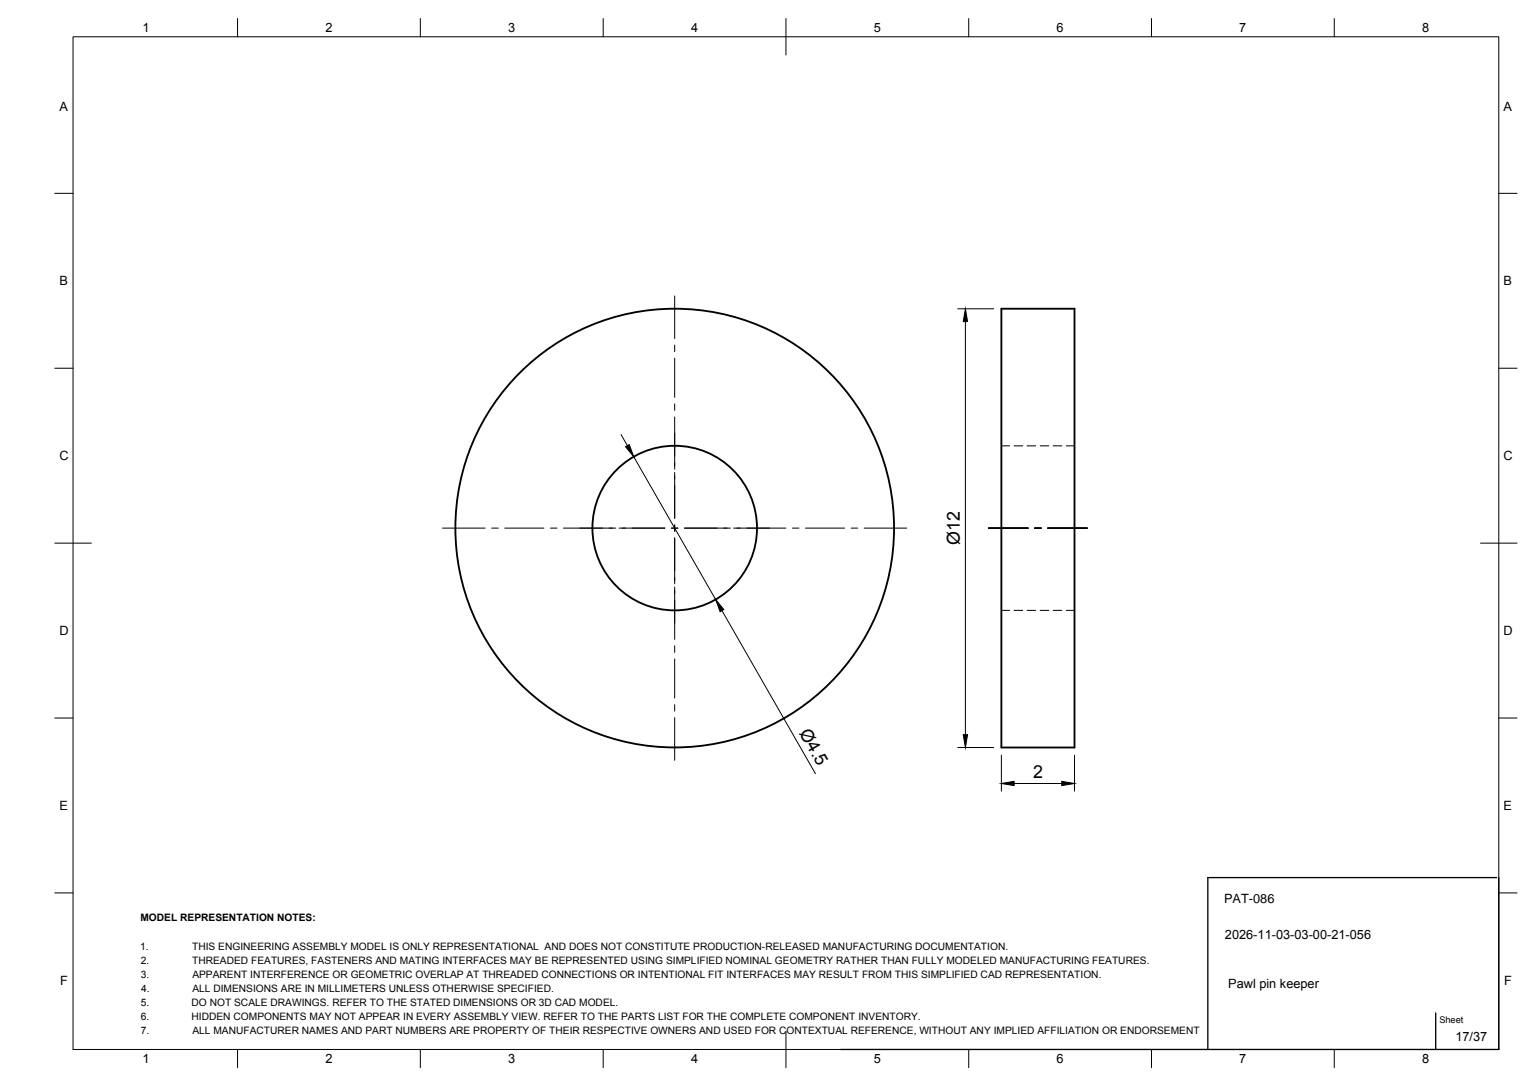
ISO-10303-21;
HEADER;
/* Generated by software containing ST-Developer
 * from STEP Tools, Inc. (www.steptools.com) 
 */

FILE_DESCRIPTION(
/* description */ ('Ratchet and pawl hand winch drum'),
/* implementation_level */ '2;1');

FILE_NAME(
/* name */ 'Pawl pin keeper.step',
/* time_stamp */ '2026-10-27T12:42:58-07:00',
/* author */ (''),
/* organization */ (''),
/* preprocessor_version */ 'ST-DEVELOPER v20.2',
/* originating_system */ 'Autodesk Translation Framework v15.17.0.0',
/* authorisation */ '');

FILE_SCHEMA (('AUTOMOTIVE_DESIGN { 1 0 10303 214 3 1 1 }'));
ENDSEC;

DATA;
#10=MECHANICAL_DESIGN_GEOMETRIC_PRESENTATION_REPRESENTATION('',(#401),#11801);
#333=SHAPE_REPRESENTATION_RELATIONSHIP('SRR','None',#11959,#367);
#367=ADVANCED_BREP_SHAPE_REPRESENTATION('',(#436),#11776);
#401=STYLED_ITEM('',(#12213),#436);
#436=MANIFOLD_SOLID_BREP('Body1',#6278);
#527=FACE_BOUND('',#1379,.T.);
#528=FACE_BOUND('',#1381,.T.);
#664=PLANE('',#6901);
#665=PLANE('',#6902);
#949=FACE_OUTER_BOUND('',#1376,.T.);
#950=FACE_OUTER_BOUND('',#1377,.T.);
#951=FACE_OUTER_BOUND('',#1378,.T.);
#952=FACE_OUTER_BOUND('',#1380,.T.);
#1376=EDGE_LOOP('',(#4691,#4692,#4693,#4694));
#1377=EDGE_LOOP('',(#4695,#4696,#4697,#4698));
#1378=EDGE_LOOP('',(#4699));
#1379=EDGE_LOOP('',(#4700));
#1380=EDGE_LOOP('',(#4701));
#1381=EDGE_LOOP('',(#4702));
#1827=LINE('',#9725,#2338);
#1828=LINE('',#9731,#2339);
#2338=VECTOR('',#7924,0.225);
#2339=VECTOR('',#7931,0.6);
#2811=CIRCLE('',#6896,0.225);
#2812=CIRCLE('',#6897,0.225);
#2813=CIRCLE('',#6899,0.6);
#2814=CIRCLE('',#6900,0.6);
#3090=VERTEX_POINT('',#9722);
#3091=VERTEX_POINT('',#9724);
#3092=VERTEX_POINT('',#9728);
#3093=VERTEX_POINT('',#9730);
#3689=EDGE_CURVE('',#3090,#3090,#2811,.T.);
#3690=EDGE_CURVE('',#3090,#3091,#1827,.T.);
#3691=EDGE_CURVE('',#3091,#3091,#2812,.T.);
#3692=EDGE_CURVE('',#3092,#3092,#2813,.T.);
#3693=EDGE_CURVE('',#3092,#3093,#1828,.T.);
#3694=EDGE_CURVE('',#3093,#3093,#2814,.T.);
#4691=ORIENTED_EDGE('',*,*,#3689,.F.);
#4692=ORIENTED_EDGE('',*,*,#3690,.T.);
#4693=ORIENTED_EDGE('',*,*,#3691,.T.);
#4694=ORIENTED_EDGE('',*,*,#3690,.F.);
#4695=ORIENTED_EDGE('',*,*,#3692,.F.);
#4696=ORIENTED_EDGE('',*,*,#3693,.T.);
#4697=ORIENTED_EDGE('',*,*,#3694,.T.);
#4698=ORIENTED_EDGE('',*,*,#3693,.F.);
#4699=ORIENTED_EDGE('',*,*,#3692,.T.);
#4700=ORIENTED_EDGE('',*,*,#3689,.T.);
#4701=ORIENTED_EDGE('',*,*,#3694,.F.);
#4702=ORIENTED_EDGE('',*,*,#3691,.F.);
#5853=CYLINDRICAL_SURFACE('',#6895,0.225);
#5854=CYLINDRICAL_SURFACE('',#6898,0.6);
#6019=ADVANCED_FACE('',(#949),#5853,.F.);
#6020=ADVANCED_FACE('',(#950),#5854,.T.);
#6021=ADVANCED_FACE('',(#951,#527),#664,.T.);
#6022=ADVANCED_FACE('',(#952,#528),#665,.F.);
#6278=CLOSED_SHELL('',(#6019,#6020,#6021,#6022));
#6894=AXIS2_PLACEMENT_3D('',#9720,#7918,#7919);
#6895=AXIS2_PLACEMENT_3D('',#9721,#7920,#7921);
#6896=AXIS2_PLACEMENT_3D('',#9723,#7922,#7923);
#6897=AXIS2_PLACEMENT_3D('',#9726,#7925,#7926);
#6898=AXIS2_PLACEMENT_3D('',#9727,#7927,#7928);
#6899=AXIS2_PLACEMENT_3D('',#9729,#7929,#7930);
#6900=AXIS2_PLACEMENT_3D('',#9732,#7932,#7933);
#6901=AXIS2_PLACEMENT_3D('',#9733,#7934,#7935);
#6902=AXIS2_PLACEMENT_3D('',#9734,#7936,#7937);
#7918=DIRECTION('axis',(0.,0.,1.));
#7919=DIRECTION('refdir',(1.,0.,0.));
#7920=DIRECTION('center_axis',(0.,1.,0.));
#7921=DIRECTION('ref_axis',(1.,0.,0.));
#7922=DIRECTION('center_axis',(0.,-1.,0.));
#7923=DIRECTION('ref_axis',(1.,0.,0.));
#7924=DIRECTION('',(0.,-1.,0.));
#7925=DIRECTION('center_axis',(0.,-1.,0.));
#7926=DIRECTION('ref_axis',(1.,0.,0.));
#7927=DIRECTION('center_axis',(0.,1.,0.));
#7928=DIRECTION('ref_axis',(1.,0.,0.));
#7929=DIRECTION('center_axis',(0.,1.,0.));
#7930=DIRECTION('ref_axis',(1.,0.,0.));
#7931=DIRECTION('',(0.,-1.,0.));
#7932=DIRECTION('center_axis',(0.,1.,0.));
#7933=DIRECTION('ref_axis',(1.,0.,0.));
#7934=DIRECTION('center_axis',(0.,1.,0.));
#7935=DIRECTION('ref_axis',(1.,0.,0.));
#7936=DIRECTION('center_axis',(0.,1.,0.));
#7937=DIRECTION('ref_axis',(1.,0.,0.));
#9720=CARTESIAN_POINT('',(0.,0.,0.));
#9721=CARTESIAN_POINT('Origin',(6.5,-2.9,10.));
#9722=CARTESIAN_POINT('',(6.275,-2.7,10.));
#9723=CARTESIAN_POINT('Origin',(6.5,-2.7,10.));
#9724=CARTESIAN_POINT('',(6.275,-2.9,10.));
#9725=CARTESIAN_POINT('',(6.275,-2.9,10.));
#9726=CARTESIAN_POINT('Origin',(6.5,-2.9,10.));
#9727=CARTESIAN_POINT('Origin',(6.5,-2.9,10.));
#9728=CARTESIAN_POINT('',(5.9,-2.7,10.));
#9729=CARTESIAN_POINT('Origin',(6.5,-2.7,10.));
#9730=CARTESIAN_POINT('',(5.9,-2.9,10.));
#9731=CARTESIAN_POINT('',(5.9,-2.9,10.));
#9732=CARTESIAN_POINT('Origin',(6.5,-2.9,10.));
#9733=CARTESIAN_POINT('Origin',(6.5,-2.7,10.));
#9734=CARTESIAN_POINT('Origin',(6.5,-2.9,10.));
#11736=UNCERTAINTY_MEASURE_WITH_UNIT(LENGTH_MEASURE(0.001),#11802,
'DISTANCE_ACCURACY_VALUE',
'Maximum model space distance between geometric entities at asserted c
onnectivities');
#11761=UNCERTAINTY_MEASURE_WITH_UNIT(LENGTH_MEASURE(0.001),#11802,
'DISTANCE_ACCURACY_VALUE',
'Maximum model space distance between geometric entities at asserted c
onnectivities');
#11776=(
GEOMETRIC_REPRESENTATION_CONTEXT(3)
GLOBAL_UNCERTAINTY_ASSIGNED_CONTEXT((#11736))
GLOBAL_UNIT_ASSIGNED_CONTEXT((#11802,#11804,#11805))
REPRESENTATION_CONTEXT('','3D')
);
#11801=(
GEOMETRIC_REPRESENTATION_CONTEXT(3)
GLOBAL_UNCERTAINTY_ASSIGNED_CONTEXT((#11761))
GLOBAL_UNIT_ASSIGNED_CONTEXT((#11802,#11804,#11805))
REPRESENTATION_CONTEXT('','3D')
);
#11802=(
LENGTH_UNIT()
NAMED_UNIT(*)
SI_UNIT(.CENTI.,.METRE.)
);
#11804=(
NAMED_UNIT(*)
PLANE_ANGLE_UNIT()
SI_UNIT($,.RADIAN.)
);
#11805=(
NAMED_UNIT(*)
SI_UNIT($,.STERADIAN.)
SOLID_ANGLE_UNIT()
);
#11820=SHAPE_DEFINITION_REPRESENTATION(#11859,#11959);
#11859=PRODUCT_DEFINITION_SHAPE('',$,#11999);
#11959=SHAPE_REPRESENTATION('',(#6894),#11776);
#11984=PRODUCT_DEFINITION_CONTEXT('part definition',#12103,'design');
#11999=PRODUCT_DEFINITION('Pawl pin keeper','Pawl pin keeper',#12038,#11984);
#12038=PRODUCT_DEFINITION_FORMATION('',$,#12119);
#12103=APPLICATION_CONTEXT(
'Core Data for Automotive Mechanical Design Process');
#12104=PRODUCT_CONTEXT('part definition',#12103,'mechanical');
#12119=PRODUCT('Pawl pin keeper','Pawl pin keeper','Pawl pin keeper',(#12104));
#12207=COLOUR_RGB('Grey',0.48,0.52,0.57);
#12208=FILL_AREA_STYLE_COLOUR('',#12207);
#12209=FILL_AREA_STYLE('',(#12208));
#12210=SURFACE_STYLE_FILL_AREA(#12209);
#12211=SURFACE_SIDE_STYLE('',(#12210));
#12212=SURFACE_STYLE_USAGE(.BOTH.,#12211);
#12213=PRESENTATION_STYLE_ASSIGNMENT((#12212));
ENDSEC;
END-ISO-10303-21;
